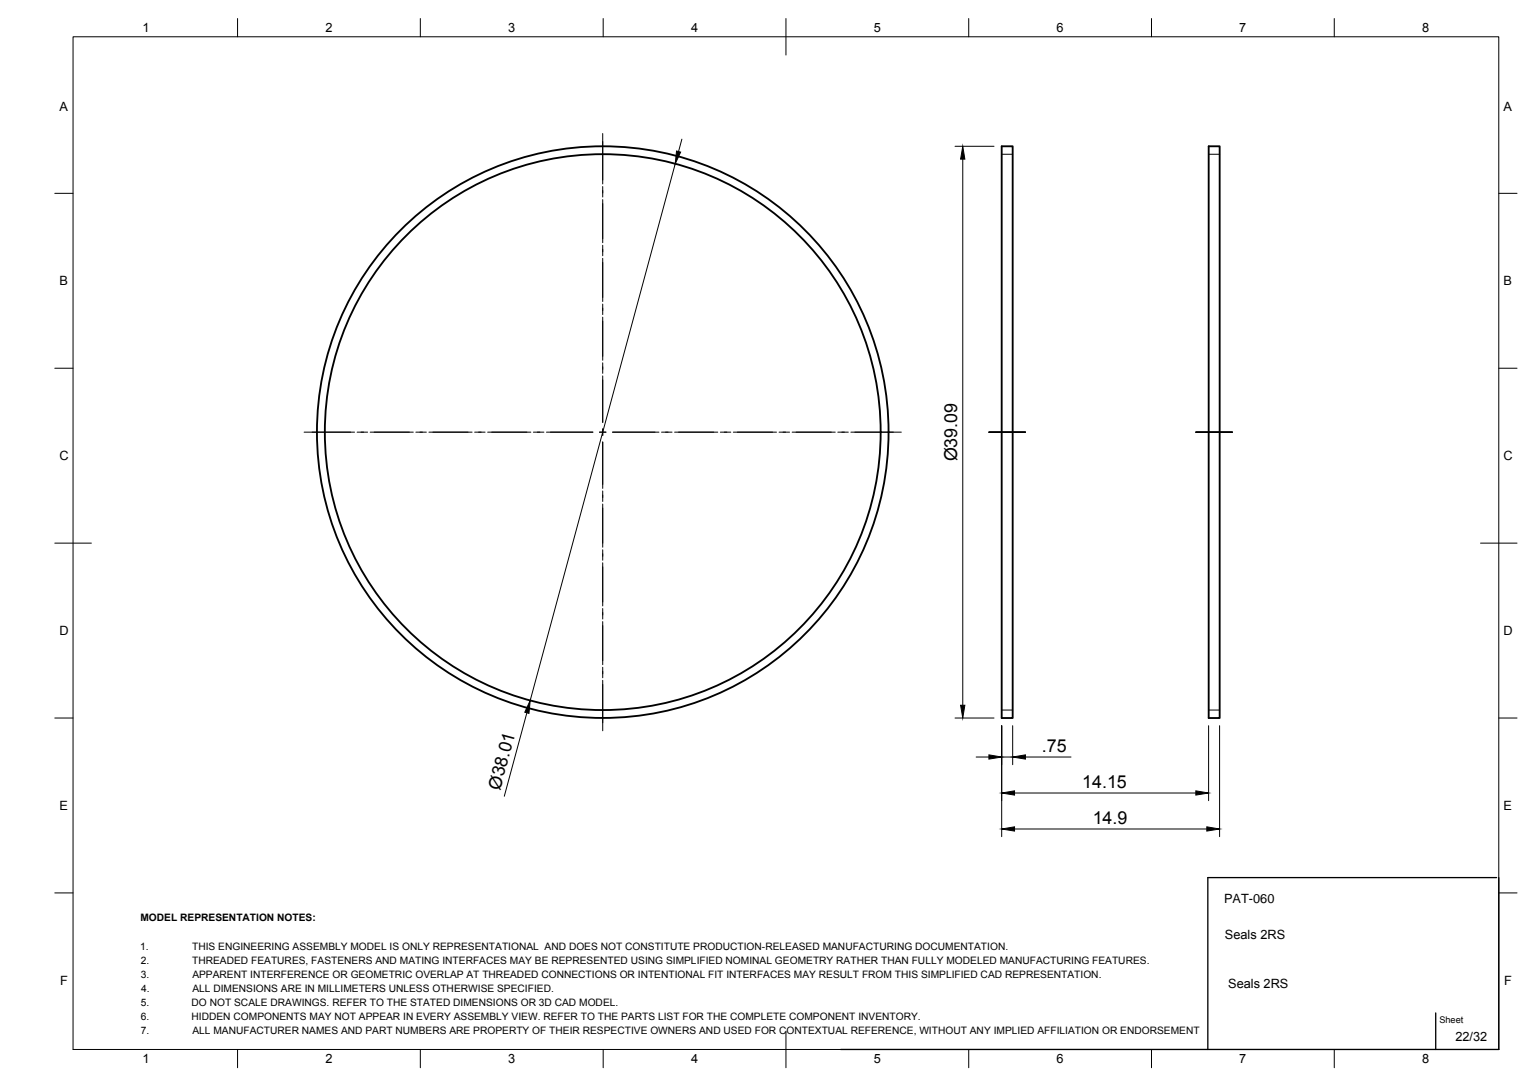
ISO-10303-21;
HEADER;
/* Generated by software containing ST-Developer
 * from STEP Tools, Inc. (www.steptools.com) 
 */

FILE_DESCRIPTION(
/* description */ ('Indexing fixture plate with plunger'),
/* implementation_level */ '2;1');

FILE_NAME(
/* name */ 'Seals 2RS.step',
/* time_stamp */ '2026-10-28T03:23:41-07:00',
/* author */ (''),
/* organization */ (''),
/* preprocessor_version */ 'ST-DEVELOPER v20.2',
/* originating_system */ 'Autodesk Translation Framework v15.17.0.0',
/* authorisation */ '');

FILE_SCHEMA (('AUTOMOTIVE_DESIGN { 1 0 10303 214 3 1 1 }'));
ENDSEC;

DATA;
#10=MECHANICAL_DESIGN_GEOMETRIC_PRESENTATION_REPRESENTATION('',(#342,#343),#10020);
#280=SHAPE_REPRESENTATION_RELATIONSHIP('SRR','None',#10155,#307);
#307=ADVANCED_BREP_SHAPE_REPRESENTATION('',(#377,#378),#10008);
#342=STYLED_ITEM('',(#10368),#377);
#343=STYLED_ITEM('',(#10368),#378);
#377=MANIFOLD_SOLID_BREP('Body1',#4597);
#378=MANIFOLD_SOLID_BREP('Body2',#4598);
#436=FACE_BOUND('',#1138,.T.);
#437=FACE_BOUND('',#1141,.T.);
#438=FACE_BOUND('',#1144,.T.);
#439=FACE_BOUND('',#1147,.T.);
#597=PLANE('',#5207);
#598=PLANE('',#5212);
#599=PLANE('',#5215);
#600=PLANE('',#5220);
#802=FACE_OUTER_BOUND('',#1137,.T.);
#803=FACE_OUTER_BOUND('',#1139,.T.);
#804=FACE_OUTER_BOUND('',#1140,.T.);
#805=FACE_OUTER_BOUND('',#1142,.T.);
#806=FACE_OUTER_BOUND('',#1143,.T.);
#807=FACE_OUTER_BOUND('',#1145,.T.);
#808=FACE_OUTER_BOUND('',#1146,.T.);
#809=FACE_OUTER_BOUND('',#1148,.T.);
#1137=EDGE_LOOP('',(#3573));
#1138=EDGE_LOOP('',(#3574));
#1139=EDGE_LOOP('',(#3575,#3576,#3577,#3578));
#1140=EDGE_LOOP('',(#3579));
#1141=EDGE_LOOP('',(#3580));
#1142=EDGE_LOOP('',(#3581,#3582,#3583,#3584));
#1143=EDGE_LOOP('',(#3585));
#1144=EDGE_LOOP('',(#3586));
#1145=EDGE_LOOP('',(#3587,#3588,#3589,#3590));
#1146=EDGE_LOOP('',(#3591));
#1147=EDGE_LOOP('',(#3592));
#1148=EDGE_LOOP('',(#3593,#3594,#3595,#3596));
#1475=LINE('',#9214,#1695);
#1476=LINE('',#9219,#1696);
#1477=LINE('',#9228,#1697);
#1478=LINE('',#9233,#1698);
#1695=VECTOR('',#6266,1.95469);
#1696=VECTOR('',#6273,1.90031);
#1697=VECTOR('',#6284,1.95469);
#1698=VECTOR('',#6291,1.90031);
#1980=CIRCLE('',#5208,1.95469);
#1981=CIRCLE('',#5209,1.90031);
#1982=CIRCLE('',#5211,1.95469);
#1983=CIRCLE('',#5213,1.90031);
#1984=CIRCLE('',#5216,1.95469);
#1985=CIRCLE('',#5217,1.90031);
#1986=CIRCLE('',#5219,1.95469);
#1987=CIRCLE('',#5221,1.90031);
#2315=VERTEX_POINT('',#9207);
#2316=VERTEX_POINT('',#9209);
#2317=VERTEX_POINT('',#9212);
#2318=VERTEX_POINT('',#9216);
#2319=VERTEX_POINT('',#9221);
#2320=VERTEX_POINT('',#9223);
#2321=VERTEX_POINT('',#9226);
#2322=VERTEX_POINT('',#9230);
#2766=EDGE_CURVE('',#2315,#2315,#1980,.T.);
#2767=EDGE_CURVE('',#2316,#2316,#1981,.T.);
#2768=EDGE_CURVE('',#2317,#2317,#1982,.T.);
#2769=EDGE_CURVE('',#2317,#2315,#1475,.T.);
#2770=EDGE_CURVE('',#2318,#2318,#1983,.T.);
#2771=EDGE_CURVE('',#2318,#2316,#1476,.T.);
#2772=EDGE_CURVE('',#2319,#2319,#1984,.T.);
#2773=EDGE_CURVE('',#2320,#2320,#1985,.T.);
#2774=EDGE_CURVE('',#2321,#2321,#1986,.T.);
#2775=EDGE_CURVE('',#2321,#2319,#1477,.T.);
#2776=EDGE_CURVE('',#2322,#2322,#1987,.T.);
#2777=EDGE_CURVE('',#2322,#2320,#1478,.T.);
#3573=ORIENTED_EDGE('',*,*,#2766,.F.);
#3574=ORIENTED_EDGE('',*,*,#2767,.T.);
#3575=ORIENTED_EDGE('',*,*,#2768,.F.);
#3576=ORIENTED_EDGE('',*,*,#2769,.T.);
#3577=ORIENTED_EDGE('',*,*,#2766,.T.);
#3578=ORIENTED_EDGE('',*,*,#2769,.F.);
#3579=ORIENTED_EDGE('',*,*,#2768,.T.);
#3580=ORIENTED_EDGE('',*,*,#2770,.F.);
#3581=ORIENTED_EDGE('',*,*,#2770,.T.);
#3582=ORIENTED_EDGE('',*,*,#2771,.T.);
#3583=ORIENTED_EDGE('',*,*,#2767,.F.);
#3584=ORIENTED_EDGE('',*,*,#2771,.F.);
#3585=ORIENTED_EDGE('',*,*,#2772,.F.);
#3586=ORIENTED_EDGE('',*,*,#2773,.T.);
#3587=ORIENTED_EDGE('',*,*,#2774,.F.);
#3588=ORIENTED_EDGE('',*,*,#2775,.T.);
#3589=ORIENTED_EDGE('',*,*,#2772,.T.);
#3590=ORIENTED_EDGE('',*,*,#2775,.F.);
#3591=ORIENTED_EDGE('',*,*,#2774,.T.);
#3592=ORIENTED_EDGE('',*,*,#2776,.F.);
#3593=ORIENTED_EDGE('',*,*,#2776,.T.);
#3594=ORIENTED_EDGE('',*,*,#2777,.T.);
#3595=ORIENTED_EDGE('',*,*,#2773,.F.);
#3596=ORIENTED_EDGE('',*,*,#2777,.F.);
#4211=CYLINDRICAL_SURFACE('',#5210,1.95469);
#4212=CYLINDRICAL_SURFACE('',#5214,1.90031);
#4213=CYLINDRICAL_SURFACE('',#5218,1.95469);
#4214=CYLINDRICAL_SURFACE('',#5222,1.90031);
#4417=ADVANCED_FACE('',(#802,#436),#597,.T.);
#4418=ADVANCED_FACE('',(#803),#4211,.T.);
#4419=ADVANCED_FACE('',(#804,#437),#598,.T.);
#4420=ADVANCED_FACE('',(#805),#4212,.F.);
#4421=ADVANCED_FACE('',(#806,#438),#599,.T.);
#4422=ADVANCED_FACE('',(#807),#4213,.T.);
#4423=ADVANCED_FACE('',(#808,#439),#600,.T.);
#4424=ADVANCED_FACE('',(#809),#4214,.F.);
#4597=CLOSED_SHELL('',(#4417,#4418,#4419,#4420));
#4598=CLOSED_SHELL('',(#4421,#4422,#4423,#4424));
#5206=AXIS2_PLACEMENT_3D('',#9205,#6254,#6255);
#5207=AXIS2_PLACEMENT_3D('',#9206,#6256,#6257);
#5208=AXIS2_PLACEMENT_3D('',#9208,#6258,#6259);
#5209=AXIS2_PLACEMENT_3D('',#9210,#6260,#6261);
#5210=AXIS2_PLACEMENT_3D('',#9211,#6262,#6263);
#5211=AXIS2_PLACEMENT_3D('',#9213,#6264,#6265);
#5212=AXIS2_PLACEMENT_3D('',#9215,#6267,#6268);
#5213=AXIS2_PLACEMENT_3D('',#9217,#6269,#6270);
#5214=AXIS2_PLACEMENT_3D('',#9218,#6271,#6272);
#5215=AXIS2_PLACEMENT_3D('',#9220,#6274,#6275);
#5216=AXIS2_PLACEMENT_3D('',#9222,#6276,#6277);
#5217=AXIS2_PLACEMENT_3D('',#9224,#6278,#6279);
#5218=AXIS2_PLACEMENT_3D('',#9225,#6280,#6281);
#5219=AXIS2_PLACEMENT_3D('',#9227,#6282,#6283);
#5220=AXIS2_PLACEMENT_3D('',#9229,#6285,#6286);
#5221=AXIS2_PLACEMENT_3D('',#9231,#6287,#6288);
#5222=AXIS2_PLACEMENT_3D('',#9232,#6289,#6290);
#6254=DIRECTION('axis',(0.,0.,1.));
#6255=DIRECTION('refdir',(1.,0.,0.));
#6256=DIRECTION('center_axis',(0.,1.,0.));
#6257=DIRECTION('ref_axis',(0.,0.,1.));
#6258=DIRECTION('center_axis',(0.,-1.,0.));
#6259=DIRECTION('ref_axis',(1.,0.,0.));
#6260=DIRECTION('center_axis',(0.,-1.,0.));
#6261=DIRECTION('ref_axis',(1.,0.,0.));
#6262=DIRECTION('center_axis',(0.,-1.,0.));
#6263=DIRECTION('ref_axis',(1.,0.,0.));
#6264=DIRECTION('center_axis',(0.,-1.,0.));
#6265=DIRECTION('ref_axis',(1.,0.,0.));
#6266=DIRECTION('',(0.,1.,0.));
#6267=DIRECTION('center_axis',(0.,-1.,0.));
#6268=DIRECTION('ref_axis',(0.,0.,-1.));
#6269=DIRECTION('center_axis',(0.,-1.,0.));
#6270=DIRECTION('ref_axis',(1.,0.,0.));
#6271=DIRECTION('center_axis',(0.,-1.,0.));
#6272=DIRECTION('ref_axis',(1.,0.,0.));
#6273=DIRECTION('',(0.,1.,0.));
#6274=DIRECTION('center_axis',(0.,1.,0.));
#6275=DIRECTION('ref_axis',(0.,0.,1.));
#6276=DIRECTION('center_axis',(0.,-1.,0.));
#6277=DIRECTION('ref_axis',(1.,0.,0.));
#6278=DIRECTION('center_axis',(0.,-1.,0.));
#6279=DIRECTION('ref_axis',(1.,0.,0.));
#6280=DIRECTION('center_axis',(0.,-1.,0.));
#6281=DIRECTION('ref_axis',(1.,0.,0.));
#6282=DIRECTION('center_axis',(0.,-1.,0.));
#6283=DIRECTION('ref_axis',(1.,0.,0.));
#6284=DIRECTION('',(0.,1.,0.));
#6285=DIRECTION('center_axis',(0.,-1.,0.));
#6286=DIRECTION('ref_axis',(0.,0.,-1.));
#6287=DIRECTION('center_axis',(0.,-1.,0.));
#6288=DIRECTION('ref_axis',(1.,0.,0.));
#6289=DIRECTION('center_axis',(0.,-1.,0.));
#6290=DIRECTION('ref_axis',(1.,0.,0.));
#6291=DIRECTION('',(0.,1.,0.));
#9205=CARTESIAN_POINT('',(0.,0.,0.));
#9206=CARTESIAN_POINT('Origin',(1.95469,0.745,0.));
#9207=CARTESIAN_POINT('',(-1.95469,0.745,-2.39380485182534E-16));
#9208=CARTESIAN_POINT('Origin',(0.,0.745,0.));
#9209=CARTESIAN_POINT('',(-1.90031,0.745,-2.32720855888771E-16));
#9210=CARTESIAN_POINT('Origin',(0.,0.745,0.));
#9211=CARTESIAN_POINT('Origin',(0.,0.7075,0.));
#9212=CARTESIAN_POINT('',(-1.95469,0.67,-2.39380485182534E-16));
#9213=CARTESIAN_POINT('Origin',(0.,0.67,0.));
#9214=CARTESIAN_POINT('',(-1.95469,0.7075,-2.39380485182534E-16));
#9215=CARTESIAN_POINT('Origin',(1.90031,0.67,0.));
#9216=CARTESIAN_POINT('',(-1.90031,0.67,-2.32720855888771E-16));
#9217=CARTESIAN_POINT('Origin',(0.,0.67,0.));
#9218=CARTESIAN_POINT('Origin',(0.,0.7075,0.));
#9219=CARTESIAN_POINT('',(-1.90031,0.7075,-2.32720855888771E-16));
#9220=CARTESIAN_POINT('Origin',(1.95469,-0.67,0.));
#9221=CARTESIAN_POINT('',(-1.95469,-0.67,-2.39380485182534E-16));
#9222=CARTESIAN_POINT('Origin',(0.,-0.67,0.));
#9223=CARTESIAN_POINT('',(-1.90031,-0.67,-2.32720855888771E-16));
#9224=CARTESIAN_POINT('Origin',(0.,-0.67,0.));
#9225=CARTESIAN_POINT('Origin',(0.,-0.7075,0.));
#9226=CARTESIAN_POINT('',(-1.95469,-0.745,-2.39380485182534E-16));
#9227=CARTESIAN_POINT('Origin',(0.,-0.745,0.));
#9228=CARTESIAN_POINT('',(-1.95469,-0.7075,-2.39380485182534E-16));
#9229=CARTESIAN_POINT('Origin',(1.90031,-0.745,0.));
#9230=CARTESIAN_POINT('',(-1.90031,-0.745,-2.32720855888771E-16));
#9231=CARTESIAN_POINT('Origin',(0.,-0.745,0.));
#9232=CARTESIAN_POINT('Origin',(0.,-0.7075,0.));
#9233=CARTESIAN_POINT('',(-1.90031,-0.7075,-2.32720855888771E-16));
#9975=UNCERTAINTY_MEASURE_WITH_UNIT(LENGTH_MEASURE(0.001),#10021,
'DISTANCE_ACCURACY_VALUE',
'Maximum model space distance between geometric entities at asserted c
onnectivities');
#9987=UNCERTAINTY_MEASURE_WITH_UNIT(LENGTH_MEASURE(0.001),#10021,
'DISTANCE_ACCURACY_VALUE',
'Maximum model space distance between geometric entities at asserted c
onnectivities');
#10008=(
GEOMETRIC_REPRESENTATION_CONTEXT(3)
GLOBAL_UNCERTAINTY_ASSIGNED_CONTEXT((#9975))
GLOBAL_UNIT_ASSIGNED_CONTEXT((#10021,#10023,#10024))
REPRESENTATION_CONTEXT('','3D')
);
#10020=(
GEOMETRIC_REPRESENTATION_CONTEXT(3)
GLOBAL_UNCERTAINTY_ASSIGNED_CONTEXT((#9987))
GLOBAL_UNIT_ASSIGNED_CONTEXT((#10021,#10023,#10024))
REPRESENTATION_CONTEXT('','3D')
);
#10021=(
LENGTH_UNIT()
NAMED_UNIT(*)
SI_UNIT(.CENTI.,.METRE.)
);
#10023=(
NAMED_UNIT(*)
PLANE_ANGLE_UNIT()
SI_UNIT($,.RADIAN.)
);
#10024=(
NAMED_UNIT(*)
SI_UNIT($,.STERADIAN.)
SOLID_ANGLE_UNIT()
);
#10045=SHAPE_DEFINITION_REPRESENTATION(#10077,#10155);
#10077=PRODUCT_DEFINITION_SHAPE('',$,#10188);
#10155=SHAPE_REPRESENTATION('',(#5206),#10008);
#10167=PRODUCT_DEFINITION_CONTEXT('part definition',#10265,'design');
#10188=PRODUCT_DEFINITION('Seals 2RS','Seals 2RS',#10220,#10167);
#10220=PRODUCT_DEFINITION_FORMATION('',$,#10287);
#10265=APPLICATION_CONTEXT(
'Core Data for Automotive Mechanical Design Process');
#10266=PRODUCT_CONTEXT('part definition',#10265,'mechanical');
#10287=PRODUCT('Seals 2RS','Seals 2RS','Seals 2RS',(#10266));
#10362=COLOUR_RGB('Grey',0.48,0.52,0.57);
#10363=FILL_AREA_STYLE_COLOUR('',#10362);
#10364=FILL_AREA_STYLE('',(#10363));
#10365=SURFACE_STYLE_FILL_AREA(#10364);
#10366=SURFACE_SIDE_STYLE('',(#10365));
#10367=SURFACE_STYLE_USAGE(.BOTH.,#10366);
#10368=PRESENTATION_STYLE_ASSIGNMENT((#10367));
ENDSEC;
END-ISO-10303-21;
